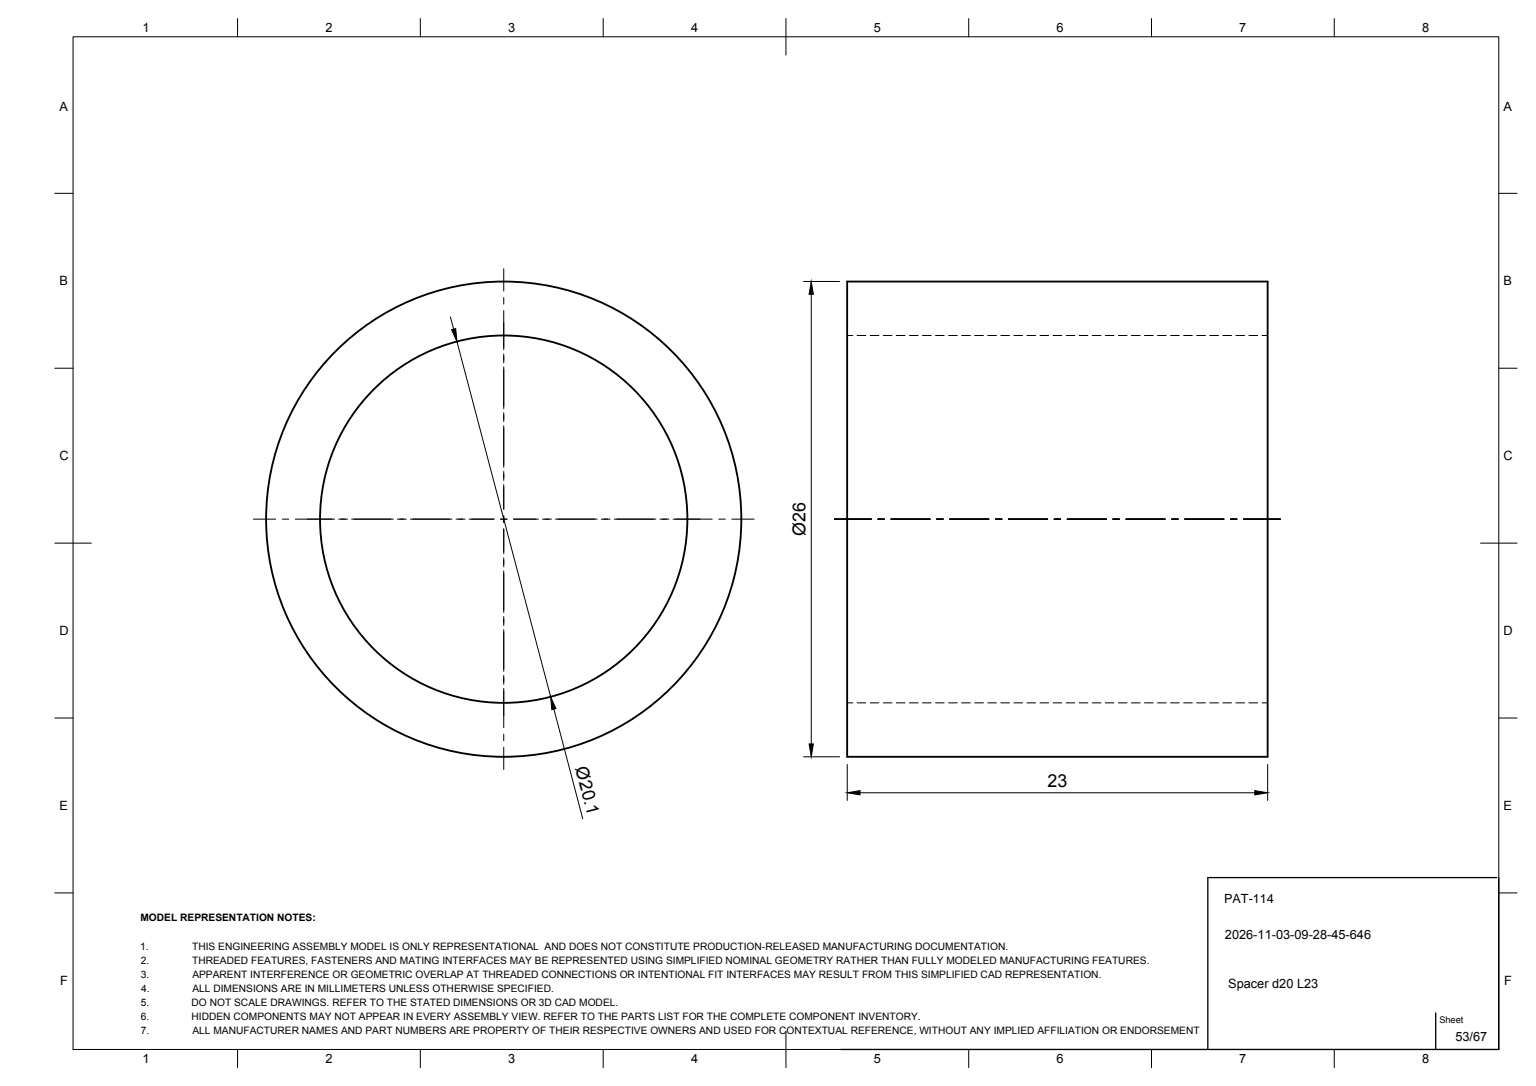
ISO-10303-21;
HEADER;
/* Generated by software containing ST-Developer
 * from STEP Tools, Inc. (www.steptools.com) 
 */

FILE_DESCRIPTION(
/* description */ ('Two-stage gear reducer in split housing'),
/* implementation_level */ '2;1');

FILE_NAME(
/* name */ 'Spacer d20 L23.step',
/* time_stamp */ '2026-10-28T03:22:31-07:00',
/* author */ (''),
/* organization */ (''),
/* preprocessor_version */ 'ST-DEVELOPER v20.2',
/* originating_system */ 'Autodesk Translation Framework v15.17.0.0',
/* authorisation */ '');

FILE_SCHEMA (('AUTOMOTIVE_DESIGN { 1 0 10303 214 3 1 1 }'));
ENDSEC;

DATA;
#10=MECHANICAL_DESIGN_GEOMETRIC_PRESENTATION_REPRESENTATION('',(#1291),#73366);
#1164=SHAPE_REPRESENTATION_RELATIONSHIP('SRR','None',#73655,#1220);
#1220=ADVANCED_BREP_SHAPE_REPRESENTATION('',(#1360),#73351);
#1291=STYLED_ITEM('',(#74002),#1360);
#1360=MANIFOLD_SOLID_BREP('Body1',#16181);
#1572=FACE_BOUND('',#3701,.T.);
#1573=FACE_BOUND('',#3703,.T.);
#1882=PLANE('',#18024);
#1883=PLANE('',#18025);
#2587=FACE_OUTER_BOUND('',#3698,.T.);
#2588=FACE_OUTER_BOUND('',#3699,.T.);
#2589=FACE_OUTER_BOUND('',#3700,.T.);
#2590=FACE_OUTER_BOUND('',#3702,.T.);
#3698=EDGE_LOOP('',(#13131,#13132,#13133,#13134));
#3699=EDGE_LOOP('',(#13135,#13136,#13137,#13138));
#3700=EDGE_LOOP('',(#13139));
#3701=EDGE_LOOP('',(#13140));
#3702=EDGE_LOOP('',(#13141));
#3703=EDGE_LOOP('',(#13142));
#4698=LINE('',#37621,#5722);
#4699=LINE('',#37627,#5723);
#5722=VECTOR('',#21516,1.005);
#5723=VECTOR('',#21523,1.3);
#6646=CIRCLE('',#18019,1.005);
#6647=CIRCLE('',#18020,1.005);
#6648=CIRCLE('',#18022,1.3);
#6649=CIRCLE('',#18023,1.3);
#7715=VERTEX_POINT('',#37618);
#7716=VERTEX_POINT('',#37620);
#7717=VERTEX_POINT('',#37624);
#7718=VERTEX_POINT('',#37626);
#9619=EDGE_CURVE('',#7715,#7715,#6646,.T.);
#9620=EDGE_CURVE('',#7715,#7716,#4698,.T.);
#9621=EDGE_CURVE('',#7716,#7716,#6647,.T.);
#9622=EDGE_CURVE('',#7717,#7717,#6648,.T.);
#9623=EDGE_CURVE('',#7717,#7718,#4699,.T.);
#9624=EDGE_CURVE('',#7718,#7718,#6649,.T.);
#13131=ORIENTED_EDGE('',*,*,#9619,.F.);
#13132=ORIENTED_EDGE('',*,*,#9620,.T.);
#13133=ORIENTED_EDGE('',*,*,#9621,.T.);
#13134=ORIENTED_EDGE('',*,*,#9620,.F.);
#13135=ORIENTED_EDGE('',*,*,#9622,.F.);
#13136=ORIENTED_EDGE('',*,*,#9623,.T.);
#13137=ORIENTED_EDGE('',*,*,#9624,.T.);
#13138=ORIENTED_EDGE('',*,*,#9623,.F.);
#13139=ORIENTED_EDGE('',*,*,#9622,.T.);
#13140=ORIENTED_EDGE('',*,*,#9619,.T.);
#13141=ORIENTED_EDGE('',*,*,#9624,.F.);
#13142=ORIENTED_EDGE('',*,*,#9621,.F.);
#15123=CYLINDRICAL_SURFACE('',#18018,1.005);
#15124=CYLINDRICAL_SURFACE('',#18021,1.3);
#15794=ADVANCED_FACE('',(#2587),#15123,.F.);
#15795=ADVANCED_FACE('',(#2588),#15124,.T.);
#15796=ADVANCED_FACE('',(#2589,#1572),#1882,.T.);
#15797=ADVANCED_FACE('',(#2590,#1573),#1883,.F.);
#16181=CLOSED_SHELL('',(#15794,#15795,#15796,#15797));
#18017=AXIS2_PLACEMENT_3D('',#37616,#21510,#21511);
#18018=AXIS2_PLACEMENT_3D('',#37617,#21512,#21513);
#18019=AXIS2_PLACEMENT_3D('',#37619,#21514,#21515);
#18020=AXIS2_PLACEMENT_3D('',#37622,#21517,#21518);
#18021=AXIS2_PLACEMENT_3D('',#37623,#21519,#21520);
#18022=AXIS2_PLACEMENT_3D('',#37625,#21521,#21522);
#18023=AXIS2_PLACEMENT_3D('',#37628,#21524,#21525);
#18024=AXIS2_PLACEMENT_3D('',#37629,#21526,#21527);
#18025=AXIS2_PLACEMENT_3D('',#37630,#21528,#21529);
#21510=DIRECTION('axis',(0.,0.,1.));
#21511=DIRECTION('refdir',(1.,0.,0.));
#21512=DIRECTION('center_axis',(0.,1.,0.));
#21513=DIRECTION('ref_axis',(1.,0.,0.));
#21514=DIRECTION('center_axis',(0.,-1.,0.));
#21515=DIRECTION('ref_axis',(1.,0.,0.));
#21516=DIRECTION('',(0.,-1.,0.));
#21517=DIRECTION('center_axis',(0.,-1.,0.));
#21518=DIRECTION('ref_axis',(1.,0.,0.));
#21519=DIRECTION('center_axis',(0.,1.,0.));
#21520=DIRECTION('ref_axis',(1.,0.,0.));
#21521=DIRECTION('center_axis',(0.,1.,0.));
#21522=DIRECTION('ref_axis',(1.,0.,0.));
#21523=DIRECTION('',(0.,-1.,0.));
#21524=DIRECTION('center_axis',(0.,1.,0.));
#21525=DIRECTION('ref_axis',(1.,0.,0.));
#21526=DIRECTION('center_axis',(0.,1.,0.));
#21527=DIRECTION('ref_axis',(1.,0.,0.));
#21528=DIRECTION('center_axis',(0.,1.,0.));
#21529=DIRECTION('ref_axis',(1.,0.,0.));
#37616=CARTESIAN_POINT('',(0.,0.,0.));
#37617=CARTESIAN_POINT('Origin',(6.,-5.3,10.));
#37618=CARTESIAN_POINT('',(4.995,-3.,10.));
#37619=CARTESIAN_POINT('Origin',(6.,-3.,10.));
#37620=CARTESIAN_POINT('',(4.995,-5.3,10.));
#37621=CARTESIAN_POINT('',(4.995,-5.3,10.));
#37622=CARTESIAN_POINT('Origin',(6.,-5.3,10.));
#37623=CARTESIAN_POINT('Origin',(6.,-5.3,10.));
#37624=CARTESIAN_POINT('',(4.7,-3.,10.));
#37625=CARTESIAN_POINT('Origin',(6.,-3.,10.));
#37626=CARTESIAN_POINT('',(4.7,-5.3,10.));
#37627=CARTESIAN_POINT('',(4.7,-5.3,10.));
#37628=CARTESIAN_POINT('Origin',(6.,-5.3,10.));
#37629=CARTESIAN_POINT('Origin',(6.,-3.,10.));
#37630=CARTESIAN_POINT('Origin',(6.,-5.3,10.));
#73287=UNCERTAINTY_MEASURE_WITH_UNIT(LENGTH_MEASURE(0.001),#73367,
'DISTANCE_ACCURACY_VALUE',
'Maximum model space distance between geometric entities at asserted c
onnectivities');
#73302=UNCERTAINTY_MEASURE_WITH_UNIT(LENGTH_MEASURE(0.001),#73367,
'DISTANCE_ACCURACY_VALUE',
'Maximum model space distance between geometric entities at asserted c
onnectivities');
#73351=(
GEOMETRIC_REPRESENTATION_CONTEXT(3)
GLOBAL_UNCERTAINTY_ASSIGNED_CONTEXT((#73287))
GLOBAL_UNIT_ASSIGNED_CONTEXT((#73367,#73369,#73370))
REPRESENTATION_CONTEXT('','3D')
);
#73366=(
GEOMETRIC_REPRESENTATION_CONTEXT(3)
GLOBAL_UNCERTAINTY_ASSIGNED_CONTEXT((#73302))
GLOBAL_UNIT_ASSIGNED_CONTEXT((#73367,#73369,#73370))
REPRESENTATION_CONTEXT('','3D')
);
#73367=(
LENGTH_UNIT()
NAMED_UNIT(*)
SI_UNIT(.CENTI.,.METRE.)
);
#73369=(
NAMED_UNIT(*)
PLANE_ANGLE_UNIT()
SI_UNIT($,.RADIAN.)
);
#73370=(
NAMED_UNIT(*)
SI_UNIT($,.STERADIAN.)
SOLID_ANGLE_UNIT()
);
#73419=SHAPE_DEFINITION_REPRESENTATION(#73552,#73655);
#73552=PRODUCT_DEFINITION_SHAPE('',$,#73719);
#73655=SHAPE_REPRESENTATION('',(#18017),#73351);
#73670=PRODUCT_DEFINITION_CONTEXT('part definition',#73861,'design');
#73719=PRODUCT_DEFINITION('Spacer d20 L23','Spacer d20 L23',#73782,#73670);
#73782=PRODUCT_DEFINITION_FORMATION('',$,#73911);
#73861=APPLICATION_CONTEXT(
'Core Data for Automotive Mechanical Design Process');
#73862=PRODUCT_CONTEXT('part definition',#73861,'mechanical');
#73911=PRODUCT('Spacer d20 L23','Spacer d20 L23','Spacer d20 L23',(#73862));
#73996=COLOUR_RGB('Off White',0.89,0.88,0.83);
#73997=FILL_AREA_STYLE_COLOUR('',#73996);
#73998=FILL_AREA_STYLE('',(#73997));
#73999=SURFACE_STYLE_FILL_AREA(#73998);
#74000=SURFACE_SIDE_STYLE('',(#73999));
#74001=SURFACE_STYLE_USAGE(.BOTH.,#74000);
#74002=PRESENTATION_STYLE_ASSIGNMENT((#74001));
ENDSEC;
END-ISO-10303-21;
